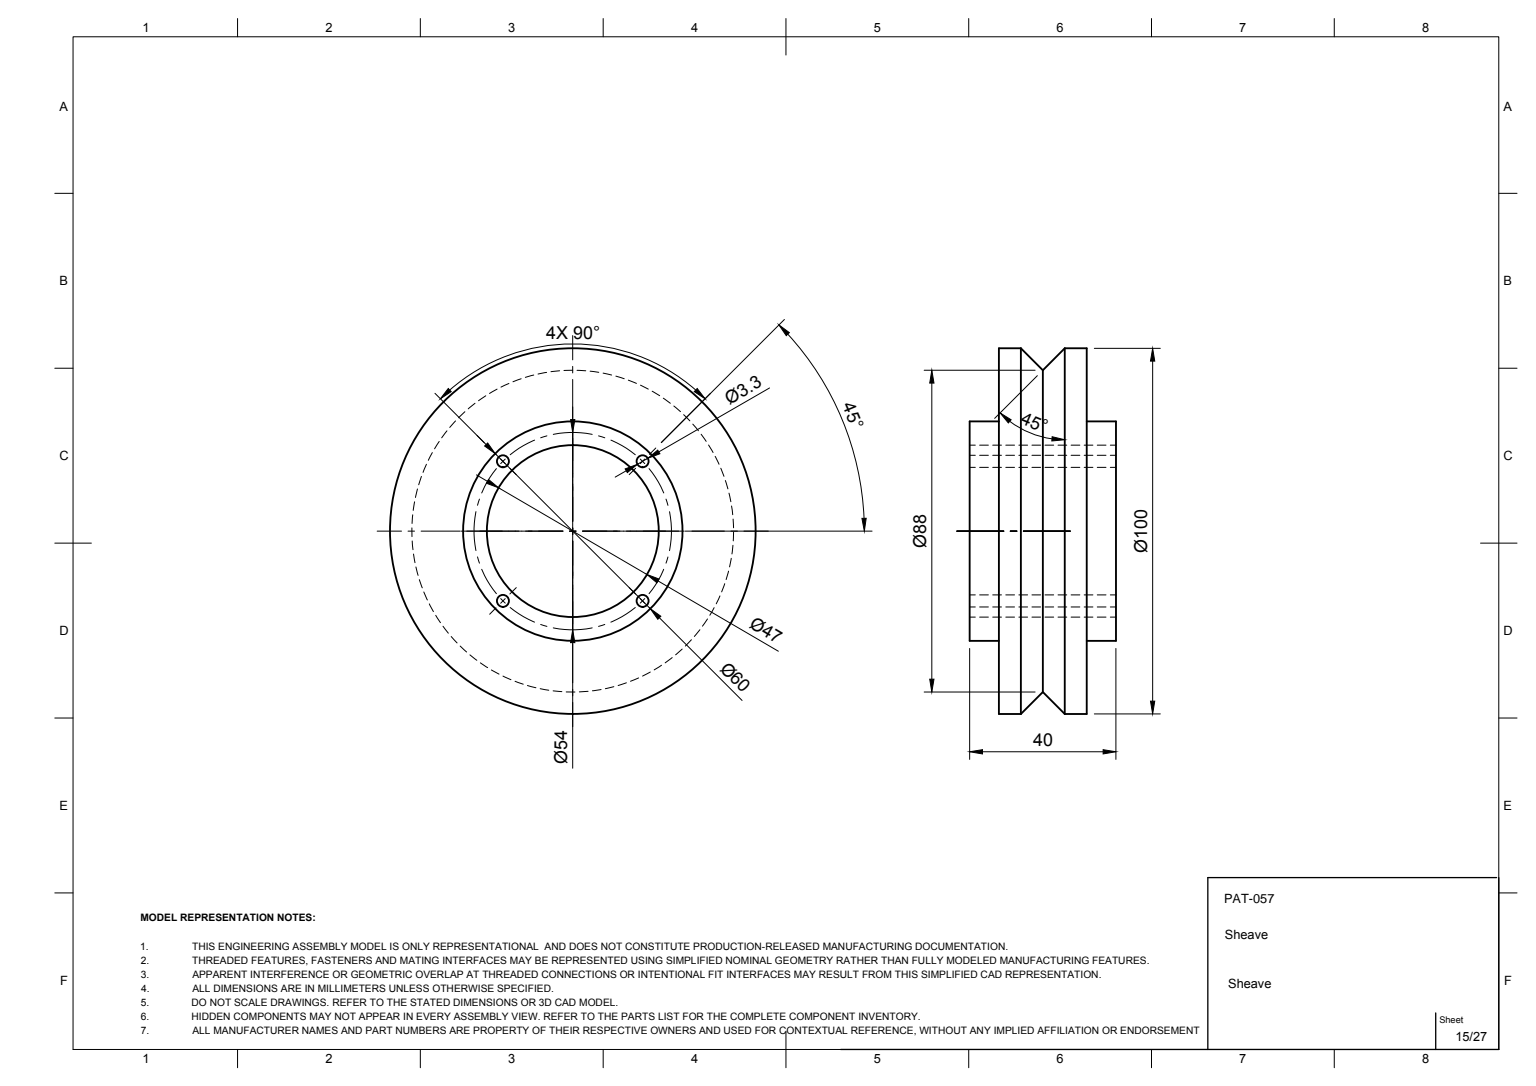
ISO-10303-21;
HEADER;
/* Generated by software containing ST-Developer
 * from STEP Tools, Inc. (www.steptools.com) 
 */

FILE_DESCRIPTION(
/* description */ ('Bearing-mounted hook block'),
/* implementation_level */ '2;1');

FILE_NAME(
/* name */ 'Sheave.step',
/* time_stamp */ '2026-10-28T22:30:11-07:00',
/* author */ (''),
/* organization */ (''),
/* preprocessor_version */ 'ST-DEVELOPER v20.2',
/* originating_system */ 'Autodesk Translation Framework v15.17.0.0',
/* authorisation */ '');

FILE_SCHEMA (('AUTOMOTIVE_DESIGN { 1 0 10303 214 3 1 1 }'));
ENDSEC;

DATA;
#10=MECHANICAL_DESIGN_GEOMETRIC_PRESENTATION_REPRESENTATION('',(#335),#7609);
#260=CONICAL_SURFACE('',#4472,4.7,0.785398163397448);
#261=CONICAL_SURFACE('',#4475,4.7,0.785398163397448);
#287=SHAPE_REPRESENTATION_RELATIONSHIP('SRR','None',#7735,#311);
#311=ADVANCED_BREP_SHAPE_REPRESENTATION('',(#365),#7595);
#335=STYLED_ITEM('',(#7924),#365);
#365=MANIFOLD_SOLID_BREP('Body1',#3933);
#512=LINE('',#6623,#742);
#513=LINE('',#6629,#743);
#514=LINE('',#6635,#744);
#515=LINE('',#6641,#745);
#516=LINE('',#6647,#746);
#517=LINE('',#6652,#747);
#518=LINE('',#6656,#748);
#519=LINE('',#6666,#749);
#520=LINE('',#6669,#750);
#521=LINE('',#6675,#751);
#522=LINE('',#6680,#752);
#742=VECTOR('',#5371,0.165);
#743=VECTOR('',#5378,0.165);
#744=VECTOR('',#5385,0.165);
#745=VECTOR('',#5392,0.165);
#746=VECTOR('',#5399,4.7);
#747=VECTOR('',#5406,4.7);
#748=VECTOR('',#5411,5.);
#749=VECTOR('',#5424,5.);
#750=VECTOR('',#5427,3.);
#751=VECTOR('',#5434,2.35);
#752=VECTOR('',#5441,3.);
#881=CYLINDRICAL_SURFACE('',#4460,0.165);
#882=CYLINDRICAL_SURFACE('',#4463,0.165);
#883=CYLINDRICAL_SURFACE('',#4466,0.165);
#884=CYLINDRICAL_SURFACE('',#4469,0.165);
#885=CYLINDRICAL_SURFACE('',#4477,5.);
#886=CYLINDRICAL_SURFACE('',#4484,5.);
#887=CYLINDRICAL_SURFACE('',#4485,3.);
#888=CYLINDRICAL_SURFACE('',#4487,2.35);
#889=CYLINDRICAL_SURFACE('',#4490,3.);
#960=FACE_BOUND('',#1395,.T.);
#961=FACE_BOUND('',#1397,.T.);
#962=FACE_BOUND('',#1403,.T.);
#963=FACE_BOUND('',#1404,.T.);
#964=FACE_BOUND('',#1405,.T.);
#965=FACE_BOUND('',#1406,.T.);
#966=FACE_BOUND('',#1407,.T.);
#967=FACE_BOUND('',#1409,.T.);
#968=FACE_BOUND('',#1410,.T.);
#969=FACE_BOUND('',#1411,.T.);
#970=FACE_BOUND('',#1412,.T.);
#971=FACE_BOUND('',#1413,.T.);
#1112=FACE_OUTER_BOUND('',#1387,.T.);
#1113=FACE_OUTER_BOUND('',#1388,.T.);
#1114=FACE_OUTER_BOUND('',#1389,.T.);
#1115=FACE_OUTER_BOUND('',#1390,.T.);
#1116=FACE_OUTER_BOUND('',#1391,.T.);
#1117=FACE_OUTER_BOUND('',#1392,.T.);
#1118=FACE_OUTER_BOUND('',#1393,.T.);
#1119=FACE_OUTER_BOUND('',#1394,.T.);
#1120=FACE_OUTER_BOUND('',#1396,.T.);
#1121=FACE_OUTER_BOUND('',#1398,.T.);
#1122=FACE_OUTER_BOUND('',#1399,.T.);
#1123=FACE_OUTER_BOUND('',#1400,.T.);
#1124=FACE_OUTER_BOUND('',#1401,.T.);
#1125=FACE_OUTER_BOUND('',#1402,.T.);
#1126=FACE_OUTER_BOUND('',#1408,.T.);
#1387=EDGE_LOOP('',(#3052,#3053,#3054,#3055));
#1388=EDGE_LOOP('',(#3056,#3057,#3058,#3059));
#1389=EDGE_LOOP('',(#3060,#3061,#3062,#3063));
#1390=EDGE_LOOP('',(#3064,#3065,#3066,#3067));
#1391=EDGE_LOOP('',(#3068,#3069,#3070,#3071));
#1392=EDGE_LOOP('',(#3072,#3073,#3074,#3075));
#1393=EDGE_LOOP('',(#3076,#3077,#3078,#3079));
#1394=EDGE_LOOP('',(#3080));
#1395=EDGE_LOOP('',(#3081));
#1396=EDGE_LOOP('',(#3082));
#1397=EDGE_LOOP('',(#3083));
#1398=EDGE_LOOP('',(#3084,#3085,#3086,#3087));
#1399=EDGE_LOOP('',(#3088,#3089,#3090,#3091));
#1400=EDGE_LOOP('',(#3092,#3093,#3094,#3095));
#1401=EDGE_LOOP('',(#3096,#3097,#3098,#3099));
#1402=EDGE_LOOP('',(#3100));
#1403=EDGE_LOOP('',(#3101));
#1404=EDGE_LOOP('',(#3102));
#1405=EDGE_LOOP('',(#3103));
#1406=EDGE_LOOP('',(#3104));
#1407=EDGE_LOOP('',(#3105));
#1408=EDGE_LOOP('',(#3106));
#1409=EDGE_LOOP('',(#3107));
#1410=EDGE_LOOP('',(#3108));
#1411=EDGE_LOOP('',(#3109));
#1412=EDGE_LOOP('',(#3110));
#1413=EDGE_LOOP('',(#3111));
#1644=CIRCLE('',#4461,0.165);
#1645=CIRCLE('',#4462,0.165);
#1646=CIRCLE('',#4464,0.165);
#1647=CIRCLE('',#4465,0.165);
#1648=CIRCLE('',#4467,0.165);
#1649=CIRCLE('',#4468,0.165);
#1650=CIRCLE('',#4470,0.165);
#1651=CIRCLE('',#4471,0.165);
#1652=CIRCLE('',#4473,4.4);
#1653=CIRCLE('',#4474,5.);
#1654=CIRCLE('',#4476,5.);
#1655=CIRCLE('',#4478,5.);
#1656=CIRCLE('',#4480,3.);
#1657=CIRCLE('',#4482,5.);
#1658=CIRCLE('',#4483,3.);
#1659=CIRCLE('',#4486,3.);
#1660=CIRCLE('',#4488,2.35);
#1661=CIRCLE('',#4489,2.35);
#1662=CIRCLE('',#4491,3.);
#1929=VERTEX_POINT('',#6620);
#1930=VERTEX_POINT('',#6622);
#1931=VERTEX_POINT('',#6626);
#1932=VERTEX_POINT('',#6628);
#1933=VERTEX_POINT('',#6632);
#1934=VERTEX_POINT('',#6634);
#1935=VERTEX_POINT('',#6638);
#1936=VERTEX_POINT('',#6640);
#1937=VERTEX_POINT('',#6644);
#1938=VERTEX_POINT('',#6646);
#1939=VERTEX_POINT('',#6650);
#1940=VERTEX_POINT('',#6654);
#1941=VERTEX_POINT('',#6658);
#1942=VERTEX_POINT('',#6661);
#1943=VERTEX_POINT('',#6663);
#1944=VERTEX_POINT('',#6668);
#1945=VERTEX_POINT('',#6672);
#1946=VERTEX_POINT('',#6674);
#1947=VERTEX_POINT('',#6678);
#2336=EDGE_CURVE('',#1929,#1929,#1644,.T.);
#2337=EDGE_CURVE('',#1929,#1930,#512,.T.);
#2338=EDGE_CURVE('',#1930,#1930,#1645,.T.);
#2339=EDGE_CURVE('',#1931,#1931,#1646,.T.);
#2340=EDGE_CURVE('',#1931,#1932,#513,.T.);
#2341=EDGE_CURVE('',#1932,#1932,#1647,.T.);
#2342=EDGE_CURVE('',#1933,#1933,#1648,.T.);
#2343=EDGE_CURVE('',#1933,#1934,#514,.T.);
#2344=EDGE_CURVE('',#1934,#1934,#1649,.T.);
#2345=EDGE_CURVE('',#1935,#1935,#1650,.T.);
#2346=EDGE_CURVE('',#1935,#1936,#515,.T.);
#2347=EDGE_CURVE('',#1936,#1936,#1651,.T.);
#2348=EDGE_CURVE('',#1937,#1937,#1652,.T.);
#2349=EDGE_CURVE('',#1937,#1938,#516,.T.);
#2350=EDGE_CURVE('',#1938,#1938,#1653,.T.);
#2351=EDGE_CURVE('',#1939,#1939,#1654,.T.);
#2352=EDGE_CURVE('',#1939,#1937,#517,.T.);
#2353=EDGE_CURVE('',#1940,#1940,#1655,.T.);
#2354=EDGE_CURVE('',#1940,#1939,#518,.T.);
#2355=EDGE_CURVE('',#1941,#1941,#1656,.T.);
#2356=EDGE_CURVE('',#1942,#1942,#1657,.T.);
#2357=EDGE_CURVE('',#1943,#1943,#1658,.T.);
#2358=EDGE_CURVE('',#1938,#1942,#519,.T.);
#2359=EDGE_CURVE('',#1943,#1944,#520,.T.);
#2360=EDGE_CURVE('',#1944,#1944,#1659,.T.);
#2361=EDGE_CURVE('',#1945,#1945,#1660,.T.);
#2362=EDGE_CURVE('',#1945,#1946,#521,.T.);
#2363=EDGE_CURVE('',#1946,#1946,#1661,.T.);
#2364=EDGE_CURVE('',#1947,#1947,#1662,.T.);
#2365=EDGE_CURVE('',#1947,#1941,#522,.T.);
#3052=ORIENTED_EDGE('',*,*,#2336,.F.);
#3053=ORIENTED_EDGE('',*,*,#2337,.T.);
#3054=ORIENTED_EDGE('',*,*,#2338,.F.);
#3055=ORIENTED_EDGE('',*,*,#2337,.F.);
#3056=ORIENTED_EDGE('',*,*,#2339,.F.);
#3057=ORIENTED_EDGE('',*,*,#2340,.T.);
#3058=ORIENTED_EDGE('',*,*,#2341,.F.);
#3059=ORIENTED_EDGE('',*,*,#2340,.F.);
#3060=ORIENTED_EDGE('',*,*,#2342,.F.);
#3061=ORIENTED_EDGE('',*,*,#2343,.T.);
#3062=ORIENTED_EDGE('',*,*,#2344,.F.);
#3063=ORIENTED_EDGE('',*,*,#2343,.F.);
#3064=ORIENTED_EDGE('',*,*,#2345,.F.);
#3065=ORIENTED_EDGE('',*,*,#2346,.T.);
#3066=ORIENTED_EDGE('',*,*,#2347,.F.);
#3067=ORIENTED_EDGE('',*,*,#2346,.F.);
#3068=ORIENTED_EDGE('',*,*,#2348,.T.);
#3069=ORIENTED_EDGE('',*,*,#2349,.T.);
#3070=ORIENTED_EDGE('',*,*,#2350,.F.);
#3071=ORIENTED_EDGE('',*,*,#2349,.F.);
#3072=ORIENTED_EDGE('',*,*,#2351,.F.);
#3073=ORIENTED_EDGE('',*,*,#2352,.T.);
#3074=ORIENTED_EDGE('',*,*,#2348,.F.);
#3075=ORIENTED_EDGE('',*,*,#2352,.F.);
#3076=ORIENTED_EDGE('',*,*,#2353,.F.);
#3077=ORIENTED_EDGE('',*,*,#2354,.T.);
#3078=ORIENTED_EDGE('',*,*,#2351,.T.);
#3079=ORIENTED_EDGE('',*,*,#2354,.F.);
#3080=ORIENTED_EDGE('',*,*,#2353,.T.);
#3081=ORIENTED_EDGE('',*,*,#2355,.F.);
#3082=ORIENTED_EDGE('',*,*,#2356,.F.);
#3083=ORIENTED_EDGE('',*,*,#2357,.F.);
#3084=ORIENTED_EDGE('',*,*,#2350,.T.);
#3085=ORIENTED_EDGE('',*,*,#2358,.T.);
#3086=ORIENTED_EDGE('',*,*,#2356,.T.);
#3087=ORIENTED_EDGE('',*,*,#2358,.F.);
#3088=ORIENTED_EDGE('',*,*,#2357,.T.);
#3089=ORIENTED_EDGE('',*,*,#2359,.T.);
#3090=ORIENTED_EDGE('',*,*,#2360,.T.);
#3091=ORIENTED_EDGE('',*,*,#2359,.F.);
#3092=ORIENTED_EDGE('',*,*,#2361,.F.);
#3093=ORIENTED_EDGE('',*,*,#2362,.T.);
#3094=ORIENTED_EDGE('',*,*,#2363,.T.);
#3095=ORIENTED_EDGE('',*,*,#2362,.F.);
#3096=ORIENTED_EDGE('',*,*,#2364,.F.);
#3097=ORIENTED_EDGE('',*,*,#2365,.T.);
#3098=ORIENTED_EDGE('',*,*,#2355,.T.);
#3099=ORIENTED_EDGE('',*,*,#2365,.F.);
#3100=ORIENTED_EDGE('',*,*,#2364,.T.);
#3101=ORIENTED_EDGE('',*,*,#2361,.T.);
#3102=ORIENTED_EDGE('',*,*,#2347,.T.);
#3103=ORIENTED_EDGE('',*,*,#2344,.T.);
#3104=ORIENTED_EDGE('',*,*,#2341,.T.);
#3105=ORIENTED_EDGE('',*,*,#2338,.T.);
#3106=ORIENTED_EDGE('',*,*,#2360,.F.);
#3107=ORIENTED_EDGE('',*,*,#2363,.F.);
#3108=ORIENTED_EDGE('',*,*,#2345,.T.);
#3109=ORIENTED_EDGE('',*,*,#2342,.T.);
#3110=ORIENTED_EDGE('',*,*,#2339,.T.);
#3111=ORIENTED_EDGE('',*,*,#2336,.T.);
#3625=PLANE('',#4479);
#3626=PLANE('',#4481);
#3627=PLANE('',#4492);
#3628=PLANE('',#4493);
#3794=ADVANCED_FACE('',(#1112),#881,.F.);
#3795=ADVANCED_FACE('',(#1113),#882,.F.);
#3796=ADVANCED_FACE('',(#1114),#883,.F.);
#3797=ADVANCED_FACE('',(#1115),#884,.F.);
#3798=ADVANCED_FACE('',(#1116),#260,.T.);
#3799=ADVANCED_FACE('',(#1117),#261,.T.);
#3800=ADVANCED_FACE('',(#1118),#885,.T.);
#3801=ADVANCED_FACE('',(#1119,#960),#3625,.T.);
#3802=ADVANCED_FACE('',(#1120,#961),#3626,.F.);
#3803=ADVANCED_FACE('',(#1121),#886,.T.);
#3804=ADVANCED_FACE('',(#1122),#887,.T.);
#3805=ADVANCED_FACE('',(#1123),#888,.F.);
#3806=ADVANCED_FACE('',(#1124),#889,.T.);
#3807=ADVANCED_FACE('',(#1125,#962,#963,#964,#965,#966),#3627,.T.);
#3808=ADVANCED_FACE('',(#1126,#967,#968,#969,#970,#971),#3628,.F.);
#3933=CLOSED_SHELL('',(#3794,#3795,#3796,#3797,#3798,#3799,#3800,#3801,
#3802,#3803,#3804,#3805,#3806,#3807,#3808));
#4459=AXIS2_PLACEMENT_3D('',#6618,#5365,#5366);
#4460=AXIS2_PLACEMENT_3D('',#6619,#5367,#5368);
#4461=AXIS2_PLACEMENT_3D('',#6621,#5369,#5370);
#4462=AXIS2_PLACEMENT_3D('',#6624,#5372,#5373);
#4463=AXIS2_PLACEMENT_3D('',#6625,#5374,#5375);
#4464=AXIS2_PLACEMENT_3D('',#6627,#5376,#5377);
#4465=AXIS2_PLACEMENT_3D('',#6630,#5379,#5380);
#4466=AXIS2_PLACEMENT_3D('',#6631,#5381,#5382);
#4467=AXIS2_PLACEMENT_3D('',#6633,#5383,#5384);
#4468=AXIS2_PLACEMENT_3D('',#6636,#5386,#5387);
#4469=AXIS2_PLACEMENT_3D('',#6637,#5388,#5389);
#4470=AXIS2_PLACEMENT_3D('',#6639,#5390,#5391);
#4471=AXIS2_PLACEMENT_3D('',#6642,#5393,#5394);
#4472=AXIS2_PLACEMENT_3D('',#6643,#5395,#5396);
#4473=AXIS2_PLACEMENT_3D('',#6645,#5397,#5398);
#4474=AXIS2_PLACEMENT_3D('',#6648,#5400,#5401);
#4475=AXIS2_PLACEMENT_3D('',#6649,#5402,#5403);
#4476=AXIS2_PLACEMENT_3D('',#6651,#5404,#5405);
#4477=AXIS2_PLACEMENT_3D('',#6653,#5407,#5408);
#4478=AXIS2_PLACEMENT_3D('',#6655,#5409,#5410);
#4479=AXIS2_PLACEMENT_3D('',#6657,#5412,#5413);
#4480=AXIS2_PLACEMENT_3D('',#6659,#5414,#5415);
#4481=AXIS2_PLACEMENT_3D('',#6660,#5416,#5417);
#4482=AXIS2_PLACEMENT_3D('',#6662,#5418,#5419);
#4483=AXIS2_PLACEMENT_3D('',#6664,#5420,#5421);
#4484=AXIS2_PLACEMENT_3D('',#6665,#5422,#5423);
#4485=AXIS2_PLACEMENT_3D('',#6667,#5425,#5426);
#4486=AXIS2_PLACEMENT_3D('',#6670,#5428,#5429);
#4487=AXIS2_PLACEMENT_3D('',#6671,#5430,#5431);
#4488=AXIS2_PLACEMENT_3D('',#6673,#5432,#5433);
#4489=AXIS2_PLACEMENT_3D('',#6676,#5435,#5436);
#4490=AXIS2_PLACEMENT_3D('',#6677,#5437,#5438);
#4491=AXIS2_PLACEMENT_3D('',#6679,#5439,#5440);
#4492=AXIS2_PLACEMENT_3D('',#6681,#5442,#5443);
#4493=AXIS2_PLACEMENT_3D('',#6682,#5444,#5445);
#5365=DIRECTION('axis',(0.,0.,1.));
#5366=DIRECTION('refdir',(1.,0.,0.));
#5367=DIRECTION('center_axis',(0.,1.,0.));
#5368=DIRECTION('ref_axis',(1.,0.,0.));
#5369=DIRECTION('center_axis',(0.,1.,0.));
#5370=DIRECTION('ref_axis',(1.,0.,0.));
#5371=DIRECTION('',(0.,1.,0.));
#5372=DIRECTION('center_axis',(0.,-1.,0.));
#5373=DIRECTION('ref_axis',(1.,0.,0.));
#5374=DIRECTION('center_axis',(0.,1.,0.));
#5375=DIRECTION('ref_axis',(1.,0.,0.));
#5376=DIRECTION('center_axis',(0.,1.,0.));
#5377=DIRECTION('ref_axis',(1.,0.,0.));
#5378=DIRECTION('',(0.,1.,0.));
#5379=DIRECTION('center_axis',(0.,-1.,0.));
#5380=DIRECTION('ref_axis',(1.,0.,0.));
#5381=DIRECTION('center_axis',(0.,1.,0.));
#5382=DIRECTION('ref_axis',(1.,0.,0.));
#5383=DIRECTION('center_axis',(0.,1.,0.));
#5384=DIRECTION('ref_axis',(1.,0.,0.));
#5385=DIRECTION('',(0.,1.,0.));
#5386=DIRECTION('center_axis',(0.,-1.,0.));
#5387=DIRECTION('ref_axis',(1.,0.,0.));
#5388=DIRECTION('center_axis',(0.,1.,0.));
#5389=DIRECTION('ref_axis',(1.,0.,0.));
#5390=DIRECTION('center_axis',(0.,1.,0.));
#5391=DIRECTION('ref_axis',(1.,0.,0.));
#5392=DIRECTION('',(0.,1.,0.));
#5393=DIRECTION('center_axis',(0.,-1.,0.));
#5394=DIRECTION('ref_axis',(1.,0.,0.));
#5395=DIRECTION('center_axis',(0.,-1.,0.));
#5396=DIRECTION('ref_axis',(1.,0.,0.));
#5397=DIRECTION('center_axis',(0.,-1.,0.));
#5398=DIRECTION('ref_axis',(1.,0.,0.));
#5399=DIRECTION('',(-0.707106781186547,-0.707106781186548,-8.65956056235493E-17));
#5400=DIRECTION('center_axis',(0.,-1.,0.));
#5401=DIRECTION('ref_axis',(1.,0.,0.));
#5402=DIRECTION('center_axis',(0.,1.,0.));
#5403=DIRECTION('ref_axis',(1.,0.,0.));
#5404=DIRECTION('center_axis',(0.,1.,0.));
#5405=DIRECTION('ref_axis',(1.,0.,0.));
#5406=DIRECTION('',(0.707106781186547,-0.707106781186548,8.65956056235493E-17));
#5407=DIRECTION('center_axis',(0.,1.,0.));
#5408=DIRECTION('ref_axis',(1.,0.,0.));
#5409=DIRECTION('center_axis',(0.,1.,0.));
#5410=DIRECTION('ref_axis',(1.,0.,0.));
#5411=DIRECTION('',(0.,-1.,0.));
#5412=DIRECTION('center_axis',(0.,1.,0.));
#5413=DIRECTION('ref_axis',(1.,0.,0.));
#5414=DIRECTION('center_axis',(0.,1.,0.));
#5415=DIRECTION('ref_axis',(1.,0.,0.));
#5416=DIRECTION('center_axis',(0.,1.,0.));
#5417=DIRECTION('ref_axis',(1.,0.,0.));
#5418=DIRECTION('center_axis',(0.,1.,0.));
#5419=DIRECTION('ref_axis',(1.,0.,0.));
#5420=DIRECTION('center_axis',(0.,-1.,0.));
#5421=DIRECTION('ref_axis',(1.,0.,0.));
#5422=DIRECTION('center_axis',(0.,1.,0.));
#5423=DIRECTION('ref_axis',(1.,0.,0.));
#5424=DIRECTION('',(0.,-1.,0.));
#5425=DIRECTION('center_axis',(0.,1.,0.));
#5426=DIRECTION('ref_axis',(1.,0.,0.));
#5427=DIRECTION('',(0.,-1.,0.));
#5428=DIRECTION('center_axis',(0.,1.,0.));
#5429=DIRECTION('ref_axis',(1.,0.,0.));
#5430=DIRECTION('center_axis',(0.,1.,0.));
#5431=DIRECTION('ref_axis',(1.,0.,0.));
#5432=DIRECTION('center_axis',(0.,-1.,0.));
#5433=DIRECTION('ref_axis',(1.,0.,0.));
#5434=DIRECTION('',(0.,-1.,0.));
#5435=DIRECTION('center_axis',(0.,-1.,0.));
#5436=DIRECTION('ref_axis',(1.,0.,0.));
#5437=DIRECTION('center_axis',(0.,1.,0.));
#5438=DIRECTION('ref_axis',(1.,0.,0.));
#5439=DIRECTION('center_axis',(0.,1.,0.));
#5440=DIRECTION('ref_axis',(1.,0.,0.));
#5441=DIRECTION('',(0.,-1.,0.));
#5442=DIRECTION('center_axis',(0.,1.,0.));
#5443=DIRECTION('ref_axis',(1.,0.,0.));
#5444=DIRECTION('center_axis',(0.,1.,0.));
#5445=DIRECTION('ref_axis',(1.,0.,0.));
#6618=CARTESIAN_POINT('',(0.,0.,0.));
#6619=CARTESIAN_POINT('Origin',(-1.90918830920368,-2.1,10.0908116907963));
#6620=CARTESIAN_POINT('',(-2.07418830920368,-2.,10.0908116907963));
#6621=CARTESIAN_POINT('Origin',(-1.90918830920368,-2.,10.0908116907963));
#6622=CARTESIAN_POINT('',(-2.07418830920368,2.,10.0908116907963));
#6623=CARTESIAN_POINT('',(-2.07418830920368,-2.1,10.0908116907963));
#6624=CARTESIAN_POINT('Origin',(-1.90918830920368,2.,10.0908116907963));
#6625=CARTESIAN_POINT('Origin',(-1.90918830920368,-2.1,13.9091883092037));
#6626=CARTESIAN_POINT('',(-2.07418830920368,-2.,13.9091883092037));
#6627=CARTESIAN_POINT('Origin',(-1.90918830920368,-2.,13.9091883092037));
#6628=CARTESIAN_POINT('',(-2.07418830920368,2.,13.9091883092037));
#6629=CARTESIAN_POINT('',(-2.07418830920368,-2.1,13.9091883092037));
#6630=CARTESIAN_POINT('Origin',(-1.90918830920368,2.,13.9091883092037));
#6631=CARTESIAN_POINT('Origin',(1.90918830920368,-2.1,13.9091883092037));
#6632=CARTESIAN_POINT('',(1.74418830920368,-2.,13.9091883092037));
#6633=CARTESIAN_POINT('Origin',(1.90918830920368,-2.,13.9091883092037));
#6634=CARTESIAN_POINT('',(1.74418830920368,2.,13.9091883092037));
#6635=CARTESIAN_POINT('',(1.74418830920368,-2.1,13.9091883092037));
#6636=CARTESIAN_POINT('Origin',(1.90918830920368,2.,13.9091883092037));
#6637=CARTESIAN_POINT('Origin',(1.90918830920368,-2.1,10.0908116907963));
#6638=CARTESIAN_POINT('',(1.74418830920368,-2.,10.0908116907963));
#6639=CARTESIAN_POINT('Origin',(1.90918830920368,-2.,10.0908116907963));
#6640=CARTESIAN_POINT('',(1.74418830920368,2.,10.0908116907963));
#6641=CARTESIAN_POINT('',(1.74418830920368,-2.1,10.0908116907963));
#6642=CARTESIAN_POINT('Origin',(1.90918830920368,2.,10.0908116907963));
#6643=CARTESIAN_POINT('Origin',(0.,-0.3,12.));
#6644=CARTESIAN_POINT('',(-4.4,4.44089209850063E-16,12.));
#6645=CARTESIAN_POINT('Origin',(0.,0.,12.));
#6646=CARTESIAN_POINT('',(-5.,-0.6,12.));
#6647=CARTESIAN_POINT('',(-4.7,-0.3,12.));
#6648=CARTESIAN_POINT('Origin',(0.,-0.6,12.));
#6649=CARTESIAN_POINT('Origin',(0.,0.3,12.));
#6650=CARTESIAN_POINT('',(-5.,0.6,12.));
#6651=CARTESIAN_POINT('Origin',(0.,0.6,12.));
#6652=CARTESIAN_POINT('',(-4.7,0.3,12.));
#6653=CARTESIAN_POINT('Origin',(0.,-1.2,12.));
#6654=CARTESIAN_POINT('',(-5.,1.2,12.));
#6655=CARTESIAN_POINT('Origin',(0.,1.2,12.));
#6656=CARTESIAN_POINT('',(-5.,-1.2,12.));
#6657=CARTESIAN_POINT('Origin',(0.,1.2,12.));
#6658=CARTESIAN_POINT('',(-3.,1.2,12.));
#6659=CARTESIAN_POINT('Origin',(0.,1.2,12.));
#6660=CARTESIAN_POINT('Origin',(0.,-1.2,12.));
#6661=CARTESIAN_POINT('',(-5.,-1.2,12.));
#6662=CARTESIAN_POINT('Origin',(0.,-1.2,12.));
#6663=CARTESIAN_POINT('',(-3.,-1.2,12.));
#6664=CARTESIAN_POINT('Origin',(0.,-1.2,12.));
#6665=CARTESIAN_POINT('Origin',(0.,-1.2,12.));
#6666=CARTESIAN_POINT('',(-5.,-1.2,12.));
#6667=CARTESIAN_POINT('Origin',(0.,-2.,12.));
#6668=CARTESIAN_POINT('',(-3.,-2.,12.));
#6669=CARTESIAN_POINT('',(-3.,-2.,12.));
#6670=CARTESIAN_POINT('Origin',(0.,-2.,12.));
#6671=CARTESIAN_POINT('Origin',(0.,-2.,12.));
#6672=CARTESIAN_POINT('',(-2.35,2.,12.));
#6673=CARTESIAN_POINT('Origin',(0.,2.,12.));
#6674=CARTESIAN_POINT('',(-2.35,-2.,12.));
#6675=CARTESIAN_POINT('',(-2.35,-2.,12.));
#6676=CARTESIAN_POINT('Origin',(0.,-2.,12.));
#6677=CARTESIAN_POINT('Origin',(0.,-2.,12.));
#6678=CARTESIAN_POINT('',(-3.,2.,12.));
#6679=CARTESIAN_POINT('Origin',(0.,2.,12.));
#6680=CARTESIAN_POINT('',(-3.,-2.,12.));
#6681=CARTESIAN_POINT('Origin',(0.,2.,12.));
#6682=CARTESIAN_POINT('Origin',(0.,-2.,12.));
#7565=UNCERTAINTY_MEASURE_WITH_UNIT(LENGTH_MEASURE(0.001),#7610,
'DISTANCE_ACCURACY_VALUE',
'Maximum model space distance between geometric entities at asserted c
onnectivities');
#7579=UNCERTAINTY_MEASURE_WITH_UNIT(LENGTH_MEASURE(0.001),#7610,
'DISTANCE_ACCURACY_VALUE',
'Maximum model space distance between geometric entities at asserted c
onnectivities');
#7595=(
GEOMETRIC_REPRESENTATION_CONTEXT(3)
GLOBAL_UNCERTAINTY_ASSIGNED_CONTEXT((#7565))
GLOBAL_UNIT_ASSIGNED_CONTEXT((#7610,#7612,#7613))
REPRESENTATION_CONTEXT('','3D')
);
#7609=(
GEOMETRIC_REPRESENTATION_CONTEXT(3)
GLOBAL_UNCERTAINTY_ASSIGNED_CONTEXT((#7579))
GLOBAL_UNIT_ASSIGNED_CONTEXT((#7610,#7612,#7613))
REPRESENTATION_CONTEXT('','3D')
);
#7610=(
LENGTH_UNIT()
NAMED_UNIT(*)
SI_UNIT(.CENTI.,.METRE.)
);
#7612=(
NAMED_UNIT(*)
PLANE_ANGLE_UNIT()
SI_UNIT($,.RADIAN.)
);
#7613=(
NAMED_UNIT(*)
SI_UNIT($,.STERADIAN.)
SOLID_ANGLE_UNIT()
);
#7629=SHAPE_DEFINITION_REPRESENTATION(#7681,#7735);
#7681=PRODUCT_DEFINITION_SHAPE('',$,#7765);
#7735=SHAPE_REPRESENTATION('',(#4459),#7595);
#7749=PRODUCT_DEFINITION_CONTEXT('part definition',#7838,'design');
#7765=PRODUCT_DEFINITION('Sheave','Sheave',#7794,#7749);
#7794=PRODUCT_DEFINITION_FORMATION('',$,#7855);
#7838=APPLICATION_CONTEXT(
'Core Data for Automotive Mechanical Design Process');
#7839=PRODUCT_CONTEXT('part definition',#7838,'mechanical');
#7855=PRODUCT('Sheave','Sheave','Sheave',(#7839));
#7918=COLOUR_RGB('Sky Blue',0.24,0.69,0.87);
#7919=FILL_AREA_STYLE_COLOUR('',#7918);
#7920=FILL_AREA_STYLE('',(#7919));
#7921=SURFACE_STYLE_FILL_AREA(#7920);
#7922=SURFACE_SIDE_STYLE('',(#7921));
#7923=SURFACE_STYLE_USAGE(.BOTH.,#7922);
#7924=PRESENTATION_STYLE_ASSIGNMENT((#7923));
ENDSEC;
END-ISO-10303-21;
